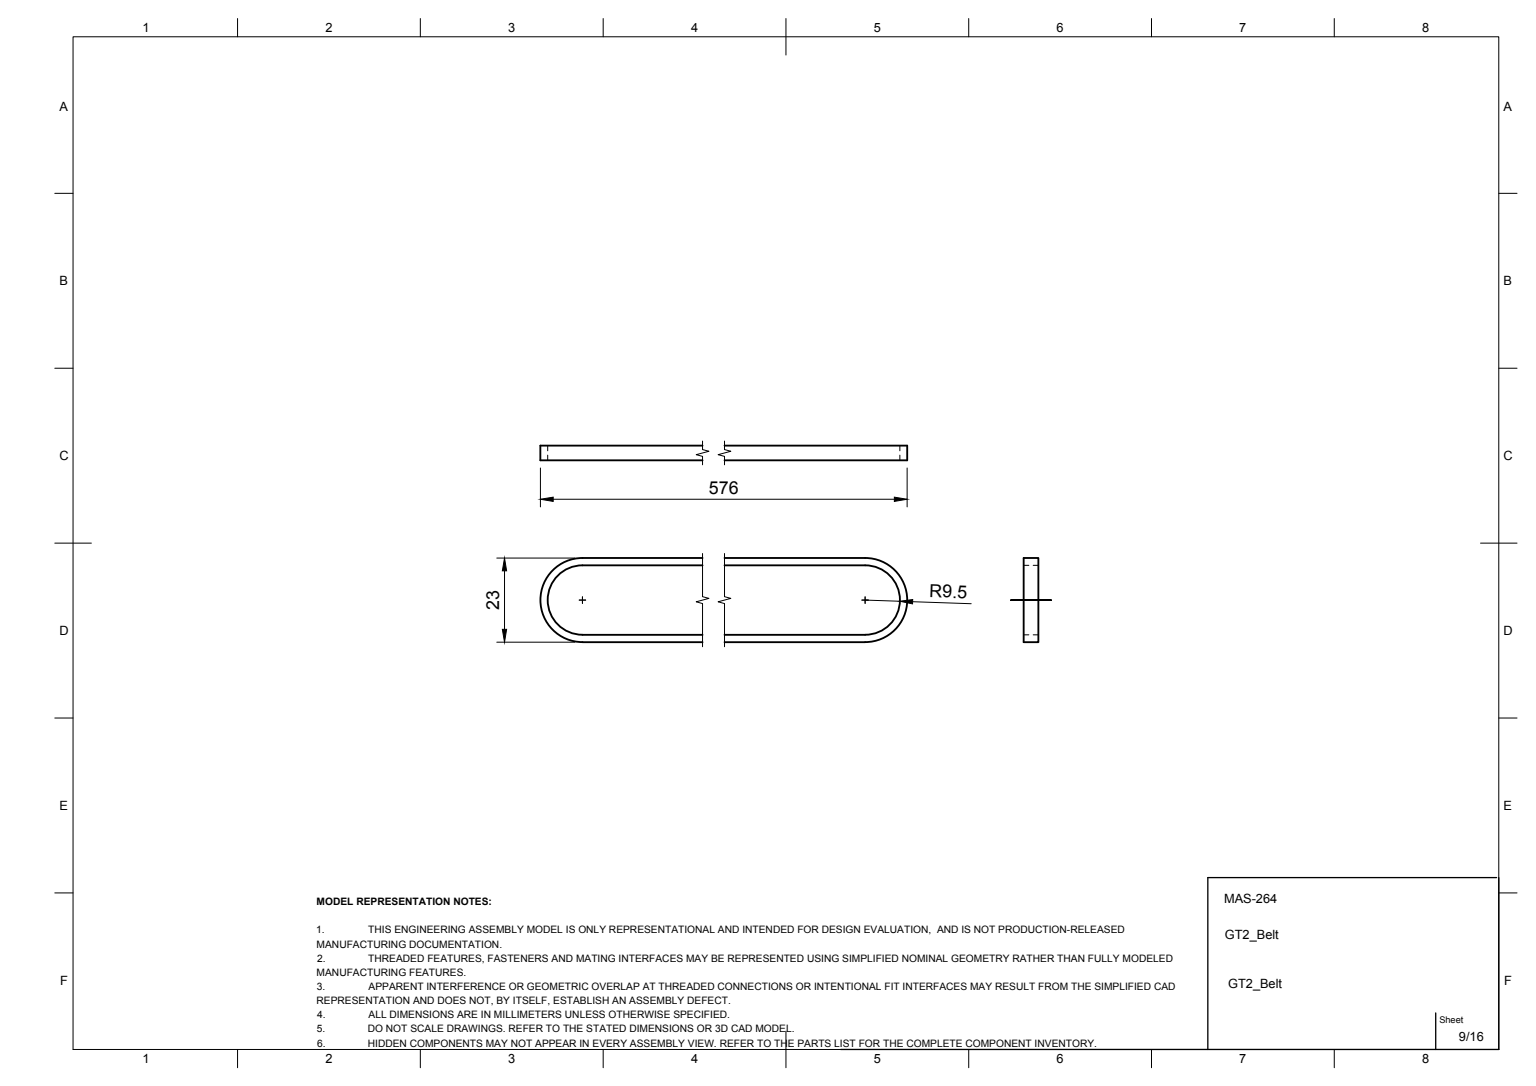
ISO-10303-21;
HEADER;
/* Generated by software containing ST-Developer
 * from STEP Tools, Inc. (www.steptools.com) 
 */

FILE_DESCRIPTION(
/* description */ (''),
/* implementation_level */ '2;1');

FILE_NAME(
/* name */ 'GT2_Belt.step',
/* time_stamp */ '2026-10-12T15:37:13-07:00',
/* author */ (''),
/* organization */ (''),
/* preprocessor_version */ 'ST-DEVELOPER v20.2',
/* originating_system */ 'Autodesk Translation Framework v15.15.0.0',
/* authorisation */ '');

FILE_SCHEMA (('AUTOMOTIVE_DESIGN { 1 0 10303 214 3 1 1 }'));
ENDSEC;

DATA;
#10=MECHANICAL_DESIGN_GEOMETRIC_PRESENTATION_REPRESENTATION('',(#354),#36460);
#115=SHAPE_REPRESENTATION_RELATIONSHIP('SRR','None',#36527,#128);
#128=ADVANCED_BREP_SHAPE_REPRESENTATION('',(#386),#36456);
#205=FACE_BOUND('',#2228,.T.);
#206=FACE_BOUND('',#2238,.T.);
#354=STYLED_ITEM('',(#36597),#386);
#386=MANIFOLD_SOLID_BREP('Body1',#11290);
#665=PLANE('',#12213);
#666=PLANE('',#12218);
#667=PLANE('',#12221);
#668=PLANE('',#12224);
#669=PLANE('',#12227);
#670=PLANE('',#12230);
#1540=FACE_OUTER_BOUND('',#2227,.T.);
#1541=FACE_OUTER_BOUND('',#2229,.T.);
#1542=FACE_OUTER_BOUND('',#2230,.T.);
#1543=FACE_OUTER_BOUND('',#2231,.T.);
#1544=FACE_OUTER_BOUND('',#2232,.T.);
#1545=FACE_OUTER_BOUND('',#2233,.T.);
#1546=FACE_OUTER_BOUND('',#2234,.T.);
#1547=FACE_OUTER_BOUND('',#2235,.T.);
#1548=FACE_OUTER_BOUND('',#2236,.T.);
#1549=FACE_OUTER_BOUND('',#2237,.T.);
#2227=EDGE_LOOP('',(#9890,#9891,#9892,#9893));
#2228=EDGE_LOOP('',(#9894,#9895,#9896,#9897));
#2229=EDGE_LOOP('',(#9898,#9899,#9900,#9901));
#2230=EDGE_LOOP('',(#9902,#9903,#9904,#9905));
#2231=EDGE_LOOP('',(#9906,#9907,#9908,#9909));
#2232=EDGE_LOOP('',(#9910,#9911,#9912,#9913));
#2233=EDGE_LOOP('',(#9914,#9915,#9916,#9917));
#2234=EDGE_LOOP('',(#9918,#9919,#9920,#9921));
#2235=EDGE_LOOP('',(#9922,#9923,#9924,#9925));
#2236=EDGE_LOOP('',(#9926,#9927,#9928,#9929));
#2237=EDGE_LOOP('',(#9930,#9931,#9932,#9933));
#2238=EDGE_LOOP('',(#9934,#9935,#9936,#9937));
#3176=LINE('',#35881,#4122);
#3177=LINE('',#35884,#4123);
#3178=LINE('',#35889,#4124);
#3179=LINE('',#35892,#4125);
#3180=LINE('',#35895,#4126);
#3181=LINE('',#35897,#4127);
#3182=LINE('',#35898,#4128);
#3183=LINE('',#35902,#4129);
#3184=LINE('',#35905,#4130);
#3185=LINE('',#35906,#4131);
#3186=LINE('',#35911,#4132);
#3187=LINE('',#35913,#4133);
#3188=LINE('',#35914,#4134);
#3189=LINE('',#35918,#4135);
#3190=LINE('',#35921,#4136);
#3191=LINE('',#35922,#4137);
#4122=VECTOR('',#14779,10.);
#4123=VECTOR('',#14782,10.);
#4124=VECTOR('',#14785,10.);
#4125=VECTOR('',#14788,10.);
#4126=VECTOR('',#14791,10.);
#4127=VECTOR('',#14792,10.);
#4128=VECTOR('',#14793,10.);
#4129=VECTOR('',#14798,10.);
#4130=VECTOR('',#14801,10.);
#4131=VECTOR('',#14802,10.);
#4132=VECTOR('',#14809,10.);
#4133=VECTOR('',#14810,10.);
#4134=VECTOR('',#14811,10.);
#4135=VECTOR('',#14816,10.);
#4136=VECTOR('',#14819,10.);
#4137=VECTOR('',#14820,10.);
#4489=CIRCLE('',#12214,11.5);
#4490=CIRCLE('',#12215,11.5);
#4491=CIRCLE('',#12216,9.5);
#4492=CIRCLE('',#12217,9.5);
#4493=CIRCLE('',#12220,9.5);
#4494=CIRCLE('',#12223,9.5);
#4495=CIRCLE('',#12226,11.5);
#4496=CIRCLE('',#12229,11.5);
#5479=VERTEX_POINT('',#35877);
#5480=VERTEX_POINT('',#35878);
#5481=VERTEX_POINT('',#35880);
#5482=VERTEX_POINT('',#35882);
#5483=VERTEX_POINT('',#35885);
#5484=VERTEX_POINT('',#35886);
#5485=VERTEX_POINT('',#35888);
#5486=VERTEX_POINT('',#35890);
#5487=VERTEX_POINT('',#35894);
#5488=VERTEX_POINT('',#35896);
#5489=VERTEX_POINT('',#35900);
#5490=VERTEX_POINT('',#35904);
#5491=VERTEX_POINT('',#35910);
#5492=VERTEX_POINT('',#35912);
#5493=VERTEX_POINT('',#35916);
#5494=VERTEX_POINT('',#35920);
#6976=EDGE_CURVE('',#5479,#5480,#4489,.T.);
#6977=EDGE_CURVE('',#5480,#5481,#3176,.T.);
#6978=EDGE_CURVE('',#5481,#5482,#4490,.T.);
#6979=EDGE_CURVE('',#5482,#5479,#3177,.T.);
#6980=EDGE_CURVE('',#5483,#5484,#4491,.T.);
#6981=EDGE_CURVE('',#5484,#5485,#3178,.T.);
#6982=EDGE_CURVE('',#5485,#5486,#4492,.T.);
#6983=EDGE_CURVE('',#5486,#5483,#3179,.T.);
#6984=EDGE_CURVE('',#5487,#5484,#3180,.T.);
#6985=EDGE_CURVE('',#5488,#5487,#3181,.T.);
#6986=EDGE_CURVE('',#5485,#5488,#3182,.T.);
#6987=EDGE_CURVE('',#5489,#5488,#4493,.T.);
#6988=EDGE_CURVE('',#5486,#5489,#3183,.T.);
#6989=EDGE_CURVE('',#5490,#5489,#3184,.T.);
#6990=EDGE_CURVE('',#5483,#5490,#3185,.T.);
#6991=EDGE_CURVE('',#5487,#5490,#4494,.T.);
#6992=EDGE_CURVE('',#5491,#5480,#3186,.T.);
#6993=EDGE_CURVE('',#5492,#5491,#3187,.T.);
#6994=EDGE_CURVE('',#5481,#5492,#3188,.T.);
#6995=EDGE_CURVE('',#5493,#5492,#4495,.T.);
#6996=EDGE_CURVE('',#5482,#5493,#3189,.T.);
#6997=EDGE_CURVE('',#5494,#5493,#3190,.T.);
#6998=EDGE_CURVE('',#5479,#5494,#3191,.T.);
#6999=EDGE_CURVE('',#5491,#5494,#4496,.T.);
#9890=ORIENTED_EDGE('',*,*,#6976,.T.);
#9891=ORIENTED_EDGE('',*,*,#6977,.T.);
#9892=ORIENTED_EDGE('',*,*,#6978,.T.);
#9893=ORIENTED_EDGE('',*,*,#6979,.T.);
#9894=ORIENTED_EDGE('',*,*,#6980,.T.);
#9895=ORIENTED_EDGE('',*,*,#6981,.T.);
#9896=ORIENTED_EDGE('',*,*,#6982,.T.);
#9897=ORIENTED_EDGE('',*,*,#6983,.T.);
#9898=ORIENTED_EDGE('',*,*,#6984,.F.);
#9899=ORIENTED_EDGE('',*,*,#6985,.F.);
#9900=ORIENTED_EDGE('',*,*,#6986,.F.);
#9901=ORIENTED_EDGE('',*,*,#6981,.F.);
#9902=ORIENTED_EDGE('',*,*,#6986,.T.);
#9903=ORIENTED_EDGE('',*,*,#6987,.F.);
#9904=ORIENTED_EDGE('',*,*,#6988,.F.);
#9905=ORIENTED_EDGE('',*,*,#6982,.F.);
#9906=ORIENTED_EDGE('',*,*,#6988,.T.);
#9907=ORIENTED_EDGE('',*,*,#6989,.F.);
#9908=ORIENTED_EDGE('',*,*,#6990,.F.);
#9909=ORIENTED_EDGE('',*,*,#6983,.F.);
#9910=ORIENTED_EDGE('',*,*,#6990,.T.);
#9911=ORIENTED_EDGE('',*,*,#6991,.F.);
#9912=ORIENTED_EDGE('',*,*,#6984,.T.);
#9913=ORIENTED_EDGE('',*,*,#6980,.F.);
#9914=ORIENTED_EDGE('',*,*,#6992,.F.);
#9915=ORIENTED_EDGE('',*,*,#6993,.F.);
#9916=ORIENTED_EDGE('',*,*,#6994,.F.);
#9917=ORIENTED_EDGE('',*,*,#6977,.F.);
#9918=ORIENTED_EDGE('',*,*,#6994,.T.);
#9919=ORIENTED_EDGE('',*,*,#6995,.F.);
#9920=ORIENTED_EDGE('',*,*,#6996,.F.);
#9921=ORIENTED_EDGE('',*,*,#6978,.F.);
#9922=ORIENTED_EDGE('',*,*,#6996,.T.);
#9923=ORIENTED_EDGE('',*,*,#6997,.F.);
#9924=ORIENTED_EDGE('',*,*,#6998,.F.);
#9925=ORIENTED_EDGE('',*,*,#6979,.F.);
#9926=ORIENTED_EDGE('',*,*,#6998,.T.);
#9927=ORIENTED_EDGE('',*,*,#6999,.F.);
#9928=ORIENTED_EDGE('',*,*,#6992,.T.);
#9929=ORIENTED_EDGE('',*,*,#6976,.F.);
#9930=ORIENTED_EDGE('',*,*,#6999,.T.);
#9931=ORIENTED_EDGE('',*,*,#6997,.T.);
#9932=ORIENTED_EDGE('',*,*,#6995,.T.);
#9933=ORIENTED_EDGE('',*,*,#6993,.T.);
#9934=ORIENTED_EDGE('',*,*,#6991,.T.);
#9935=ORIENTED_EDGE('',*,*,#6989,.T.);
#9936=ORIENTED_EDGE('',*,*,#6987,.T.);
#9937=ORIENTED_EDGE('',*,*,#6985,.T.);
#10599=CYLINDRICAL_SURFACE('',#12219,9.5);
#10600=CYLINDRICAL_SURFACE('',#12222,9.5);
#10601=CYLINDRICAL_SURFACE('',#12225,11.5);
#10602=CYLINDRICAL_SURFACE('',#12228,11.5);
#11161=ADVANCED_FACE('',(#1540,#205),#665,.F.);
#11162=ADVANCED_FACE('',(#1541),#666,.T.);
#11163=ADVANCED_FACE('',(#1542),#10599,.F.);
#11164=ADVANCED_FACE('',(#1543),#667,.T.);
#11165=ADVANCED_FACE('',(#1544),#10600,.F.);
#11166=ADVANCED_FACE('',(#1545),#668,.T.);
#11167=ADVANCED_FACE('',(#1546),#10601,.T.);
#11168=ADVANCED_FACE('',(#1547),#669,.T.);
#11169=ADVANCED_FACE('',(#1548),#10602,.T.);
#11170=ADVANCED_FACE('',(#1549,#206),#670,.T.);
#11290=CLOSED_SHELL('',(#11161,#11162,#11163,#11164,#11165,#11166,#11167,
#11168,#11169,#11170));
#12212=AXIS2_PLACEMENT_3D('',#35875,#14773,#14774);
#12213=AXIS2_PLACEMENT_3D('',#35876,#14775,#14776);
#12214=AXIS2_PLACEMENT_3D('',#35879,#14777,#14778);
#12215=AXIS2_PLACEMENT_3D('',#35883,#14780,#14781);
#12216=AXIS2_PLACEMENT_3D('',#35887,#14783,#14784);
#12217=AXIS2_PLACEMENT_3D('',#35891,#14786,#14787);
#12218=AXIS2_PLACEMENT_3D('',#35893,#14789,#14790);
#12219=AXIS2_PLACEMENT_3D('',#35899,#14794,#14795);
#12220=AXIS2_PLACEMENT_3D('',#35901,#14796,#14797);
#12221=AXIS2_PLACEMENT_3D('',#35903,#14799,#14800);
#12222=AXIS2_PLACEMENT_3D('',#35907,#14803,#14804);
#12223=AXIS2_PLACEMENT_3D('',#35908,#14805,#14806);
#12224=AXIS2_PLACEMENT_3D('',#35909,#14807,#14808);
#12225=AXIS2_PLACEMENT_3D('',#35915,#14812,#14813);
#12226=AXIS2_PLACEMENT_3D('',#35917,#14814,#14815);
#12227=AXIS2_PLACEMENT_3D('',#35919,#14817,#14818);
#12228=AXIS2_PLACEMENT_3D('',#35923,#14821,#14822);
#12229=AXIS2_PLACEMENT_3D('',#35924,#14823,#14824);
#12230=AXIS2_PLACEMENT_3D('',#35925,#14825,#14826);
#14773=DIRECTION('axis',(0.,0.,1.));
#14774=DIRECTION('refdir',(1.,0.,0.));
#14775=DIRECTION('center_axis',(0.,0.,1.));
#14776=DIRECTION('ref_axis',(1.,0.,0.));
#14777=DIRECTION('center_axis',(0.,0.,-1.));
#14778=DIRECTION('ref_axis',(-1.,-1.54465812121761E-15,0.));
#14779=DIRECTION('',(0.,1.,0.));
#14780=DIRECTION('center_axis',(0.,0.,-1.));
#14781=DIRECTION('ref_axis',(1.,0.,0.));
#14782=DIRECTION('',(1.00381828627953E-18,-1.,0.));
#14783=DIRECTION('center_axis',(0.,0.,1.));
#14784=DIRECTION('ref_axis',(-1.,-1.86984930463184E-15,0.));
#14785=DIRECTION('',(0.,1.,0.));
#14786=DIRECTION('center_axis',(0.,0.,1.));
#14787=DIRECTION('ref_axis',(1.,0.,0.));
#14788=DIRECTION('',(0.,-1.,0.));
#14789=DIRECTION('center_axis',(-1.,0.,0.));
#14790=DIRECTION('ref_axis',(0.,-1.,0.));
#14791=DIRECTION('',(0.,0.,-1.));
#14792=DIRECTION('',(0.,-1.,0.));
#14793=DIRECTION('',(0.,0.,1.));
#14794=DIRECTION('center_axis',(0.,0.,1.));
#14795=DIRECTION('ref_axis',(1.,0.,0.));
#14796=DIRECTION('center_axis',(0.,0.,-1.));
#14797=DIRECTION('ref_axis',(1.,0.,0.));
#14798=DIRECTION('',(0.,0.,1.));
#14799=DIRECTION('center_axis',(1.,0.,0.));
#14800=DIRECTION('ref_axis',(0.,1.,0.));
#14801=DIRECTION('',(0.,1.,0.));
#14802=DIRECTION('',(0.,0.,1.));
#14803=DIRECTION('center_axis',(0.,0.,1.));
#14804=DIRECTION('ref_axis',(-1.,-1.86984930463184E-15,0.));
#14805=DIRECTION('center_axis',(0.,0.,-1.));
#14806=DIRECTION('ref_axis',(-1.,-1.86984930463184E-15,0.));
#14807=DIRECTION('center_axis',(-1.,0.,0.));
#14808=DIRECTION('ref_axis',(0.,-1.,0.));
#14809=DIRECTION('',(0.,0.,-1.));
#14810=DIRECTION('',(0.,-1.,0.));
#14811=DIRECTION('',(0.,0.,1.));
#14812=DIRECTION('center_axis',(0.,0.,1.));
#14813=DIRECTION('ref_axis',(1.,0.,0.));
#14814=DIRECTION('center_axis',(0.,0.,1.));
#14815=DIRECTION('ref_axis',(1.,0.,0.));
#14816=DIRECTION('',(0.,0.,1.));
#14817=DIRECTION('center_axis',(1.,1.00381828627953E-18,0.));
#14818=DIRECTION('ref_axis',(-1.00381828627953E-18,1.,0.));
#14819=DIRECTION('',(-1.00381828627953E-18,1.,0.));
#14820=DIRECTION('',(0.,0.,1.));
#14821=DIRECTION('center_axis',(0.,0.,1.));
#14822=DIRECTION('ref_axis',(-1.,-1.54465812121761E-15,0.));
#14823=DIRECTION('center_axis',(0.,0.,1.));
#14824=DIRECTION('ref_axis',(-1.,-1.54465812121761E-15,0.));
#14825=DIRECTION('center_axis',(0.,0.,1.));
#14826=DIRECTION('ref_axis',(1.,0.,0.));
#35875=CARTESIAN_POINT('',(0.,0.,0.));
#35876=CARTESIAN_POINT('Origin',(-9.99999999999996,243.556498641762,-1.25799999999979));
#35877=CARTESIAN_POINT('',(1.50000000000004,-32.9435013582377,-1.25799999999979));
#35878=CARTESIAN_POINT('',(-21.5,-32.9435013582377,-1.25799999999979));
#35879=CARTESIAN_POINT('Origin',(-9.99999999999996,-32.9435013582377,-1.25799999999979));
#35880=CARTESIAN_POINT('',(-21.5,520.056498641762,-1.25799999999979));
#35881=CARTESIAN_POINT('',(-21.5,520.056498641762,-1.25799999999979));
#35882=CARTESIAN_POINT('',(1.50000000000004,520.056498641762,-1.25799999999979));
#35883=CARTESIAN_POINT('Origin',(-9.99999999999996,520.056498641762,-1.25799999999979));
#35884=CARTESIAN_POINT('',(1.50000000000004,-32.9435013582377,-1.25799999999979));
#35885=CARTESIAN_POINT('',(-19.5,-32.9435013582377,-1.25799999999979));
#35886=CARTESIAN_POINT('',(-0.499999999999963,-32.9435013582377,-1.25799999999979));
#35887=CARTESIAN_POINT('Origin',(-9.99999999999996,-32.9435013582377,-1.25799999999979));
#35888=CARTESIAN_POINT('',(-0.499999999999963,520.056498641762,-1.25799999999979));
#35889=CARTESIAN_POINT('',(-0.499999999999963,-32.9435013582377,-1.25799999999979));
#35890=CARTESIAN_POINT('',(-19.5,520.056498641762,-1.25799999999979));
#35891=CARTESIAN_POINT('Origin',(-9.99999999999996,520.056498641762,-1.25799999999979));
#35892=CARTESIAN_POINT('',(-19.5,520.056498641762,-1.25799999999979));
#35893=CARTESIAN_POINT('Origin',(-0.499999999999963,520.056498641762,0.742000000000206));
#35894=CARTESIAN_POINT('',(-0.499999999999963,-32.9435013582377,2.74200000000021));
#35895=CARTESIAN_POINT('',(-0.499999999999963,-32.9435013582377,0.742000000000206));
#35896=CARTESIAN_POINT('',(-0.499999999999963,520.056498641762,2.74200000000021));
#35897=CARTESIAN_POINT('',(-0.499999999999963,-32.9435013582377,2.74200000000021));
#35898=CARTESIAN_POINT('',(-0.499999999999963,520.056498641762,0.742000000000206));
#35899=CARTESIAN_POINT('Origin',(-9.99999999999996,520.056498641762,0.742000000000206));
#35900=CARTESIAN_POINT('',(-19.5,520.056498641762,2.74200000000021));
#35901=CARTESIAN_POINT('Origin',(-9.99999999999996,520.056498641762,2.74200000000021));
#35902=CARTESIAN_POINT('',(-19.5,520.056498641762,0.742000000000206));
#35903=CARTESIAN_POINT('Origin',(-19.5,-32.9435013582377,0.742000000000206));
#35904=CARTESIAN_POINT('',(-19.5,-32.9435013582377,2.74200000000021));
#35905=CARTESIAN_POINT('',(-19.5,520.056498641762,2.74200000000021));
#35906=CARTESIAN_POINT('',(-19.5,-32.9435013582377,0.742000000000206));
#35907=CARTESIAN_POINT('Origin',(-9.99999999999996,-32.9435013582377,0.742000000000206));
#35908=CARTESIAN_POINT('Origin',(-9.99999999999996,-32.9435013582377,2.74200000000021));
#35909=CARTESIAN_POINT('Origin',(-21.5,520.056498641762,0.742000000000206));
#35910=CARTESIAN_POINT('',(-21.5,-32.9435013582377,2.74200000000021));
#35911=CARTESIAN_POINT('',(-21.5,-32.9435013582377,0.742000000000206));
#35912=CARTESIAN_POINT('',(-21.5,520.056498641762,2.74200000000021));
#35913=CARTESIAN_POINT('',(-21.5,520.056498641762,2.74200000000021));
#35914=CARTESIAN_POINT('',(-21.5,520.056498641762,0.742000000000206));
#35915=CARTESIAN_POINT('Origin',(-9.99999999999996,520.056498641762,0.742000000000206));
#35916=CARTESIAN_POINT('',(1.50000000000004,520.056498641762,2.74200000000021));
#35917=CARTESIAN_POINT('Origin',(-9.99999999999996,520.056498641762,2.74200000000021));
#35918=CARTESIAN_POINT('',(1.50000000000004,520.056498641762,0.742000000000206));
#35919=CARTESIAN_POINT('Origin',(1.50000000000004,-32.9435013582377,0.742000000000206));
#35920=CARTESIAN_POINT('',(1.50000000000004,-32.9435013582377,2.74200000000021));
#35921=CARTESIAN_POINT('',(1.50000000000004,-32.9435013582377,2.74200000000021));
#35922=CARTESIAN_POINT('',(1.50000000000004,-32.9435013582377,0.742000000000206));
#35923=CARTESIAN_POINT('Origin',(-9.99999999999996,-32.9435013582377,0.742000000000206));
#35924=CARTESIAN_POINT('Origin',(-9.99999999999996,-32.9435013582377,2.74200000000021));
#35925=CARTESIAN_POINT('Origin',(-9.99999999999996,243.556498641762,2.74200000000021));
#36440=UNCERTAINTY_MEASURE_WITH_UNIT(LENGTH_MEASURE(0.01),#36461,
'DISTANCE_ACCURACY_VALUE',
'Maximum model space distance between geometric entities at asserted c
onnectivities');
#36444=UNCERTAINTY_MEASURE_WITH_UNIT(LENGTH_MEASURE(0.01),#36461,
'DISTANCE_ACCURACY_VALUE',
'Maximum model space distance between geometric entities at asserted c
onnectivities');
#36456=(
GEOMETRIC_REPRESENTATION_CONTEXT(3)
GLOBAL_UNCERTAINTY_ASSIGNED_CONTEXT((#36440))
GLOBAL_UNIT_ASSIGNED_CONTEXT((#36461,#36463,#36464))
REPRESENTATION_CONTEXT('','3D')
);
#36460=(
GEOMETRIC_REPRESENTATION_CONTEXT(3)
GLOBAL_UNCERTAINTY_ASSIGNED_CONTEXT((#36444))
GLOBAL_UNIT_ASSIGNED_CONTEXT((#36461,#36463,#36464))
REPRESENTATION_CONTEXT('','3D')
);
#36461=(
LENGTH_UNIT()
NAMED_UNIT(*)
SI_UNIT(.MILLI.,.METRE.)
);
#36463=(
NAMED_UNIT(*)
PLANE_ANGLE_UNIT()
SI_UNIT($,.RADIAN.)
);
#36464=(
NAMED_UNIT(*)
SI_UNIT($,.STERADIAN.)
SOLID_ANGLE_UNIT()
);
#36476=SHAPE_DEFINITION_REPRESENTATION(#36496,#36527);
#36496=PRODUCT_DEFINITION_SHAPE('',$,#36543);
#36527=SHAPE_REPRESENTATION('',(#12212),#36456);
#36531=PRODUCT_DEFINITION_CONTEXT('part definition',#36578,'design');
#36543=PRODUCT_DEFINITION('GT2_Belt','GT2_Belt',#36558,#36531);
#36558=PRODUCT_DEFINITION_FORMATION('',$,#36591);
#36578=APPLICATION_CONTEXT(
'Core Data for Automotive Mechanical Design Process');
#36579=PRODUCT_CONTEXT('part definition',#36578,'mechanical');
#36591=PRODUCT('GT2_Belt','GT2_Belt',$,(#36579));
#36597=PRESENTATION_STYLE_ASSIGNMENT((#36602));
#36602=SURFACE_STYLE_USAGE(.BOTH.,#36607);
#36607=SURFACE_SIDE_STYLE('',(#36612));
#36612=SURFACE_STYLE_FILL_AREA(#36617);
#36617=FILL_AREA_STYLE('Opaque(39,39,39)',(#36622));
#36622=FILL_AREA_STYLE_COLOUR('Opaque(39,39,39)',#36627);
#36627=COLOUR_RGB('Opaque(39,39,39)', 0.31764706, 0.68627451, 0.89019608);
ENDSEC;
END-ISO-10303-21;
